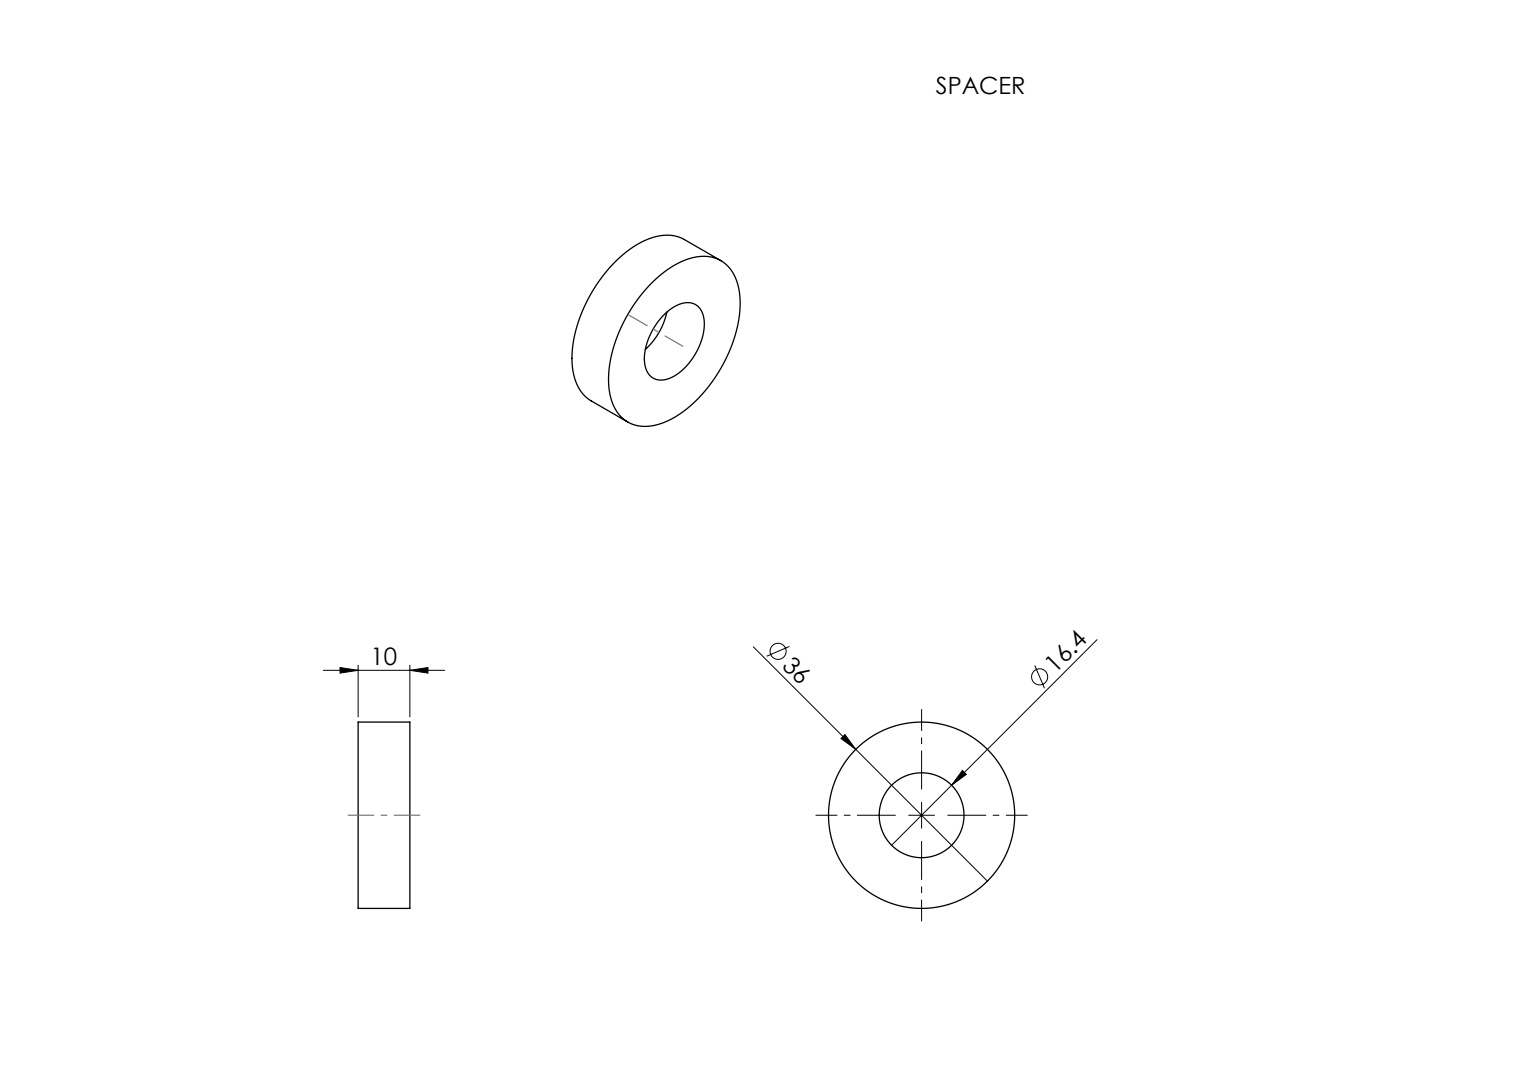
ISO-10303-21;
HEADER;
FILE_DESCRIPTION (('STEP AP214'),
    '1' );
FILE_NAME ('spacer.step',
    '2026-10-08T13:22:57',
    ( '' ),
    ( '' ),
    'SwSTEP 2.0',
    'SolidWorks 2026',
    '' );
FILE_SCHEMA (( 'AUTOMOTIVE_DESIGN' ));
ENDSEC;

DATA;
#27=LINE ( 'NONE', #8664, #6923 ) ;
#42=ORIENTED_EDGE ( 'NONE', *, *, #8056, .T. ) ;
#95=DIRECTION ( 'NONE',  ( 0.000000000000000000, 0.000000000000000000, 1.000000000000000000 ) ) ;
#147=MANIFOLD_SOLID_BREP ( 'Revolve1', #1849 ) ;
#192=( GEOMETRIC_REPRESENTATION_CONTEXT ( 3 ) GLOBAL_UNCERTAINTY_ASSIGNED_CONTEXT ( ( #920 ) ) GLOBAL_UNIT_ASSIGNED_CONTEXT ( ( #9393, #2545, #4632 ) ) REPRESENTATION_CONTEXT ( 'NONE', 'WORKASPACE' ) );
#245=CARTESIAN_POINT ( 'NONE',  ( 0.000000000000000000, 0.000000000000000000, 0.000000000000000000 ) ) ;
#270=( NAMED_UNIT ( * ) SI_UNIT ( $, .STERADIAN. ) SOLID_ANGLE_UNIT ( ) );
#321=ORIENTED_EDGE ( 'NONE', *, *, #2438, .F. ) ;
#336=AXIS2_PLACEMENT_3D ( 'NONE', #4011, #10212, #2306 ) ;
#339=AXIS2_PLACEMENT_3D ( 'NONE', #8130, #857, #5651 ) ;
#372=DIRECTION ( 'NONE',  ( -1.000000000000000000, 0.000000000000000000, -0.000000000000000000 ) ) ;
#398=UNCERTAINTY_MEASURE_WITH_UNIT (LENGTH_MEASURE( 1.000000000000000082E-05 ), #6272, 'distance_accuracy_value', 'NONE');
#440=DIRECTION ( 'NONE',  ( -1.000000000000000000, -0.000000000000000000, -0.000000000000000000 ) ) ;
#540=ORIENTED_EDGE ( 'NONE', *, *, #3932, .F. ) ;
#600=DIRECTION ( 'NONE',  ( -1.000000000000000000, -0.000000000000000000, -0.000000000000000000 ) ) ;
#614=SURFACE_STYLE_FILL_AREA ( #1388 ) ;
#808=EDGE_LOOP ( 'NONE', ( #8183, #7478, #5542, #1198 ) ) ;
#857=DIRECTION ( 'NONE',  ( -1.000000000000000000, -0.000000000000000000, -0.000000000000000000 ) ) ;
#920=UNCERTAINTY_MEASURE_WITH_UNIT (LENGTH_MEASURE( 1.000000000000000082E-05 ), #9393, 'distance_accuracy_value', 'NONE');
#1028=STYLED_ITEM ( 'NONE', ( #10063 ), #147 ) ;
#1052=DIRECTION ( 'NONE',  ( 0.000000000000000000, 0.000000000000000000, 1.000000000000000000 ) ) ;
#1099=DIRECTION ( 'NONE',  ( -1.000000000000000000, -0.000000000000000000, -0.000000000000000000 ) ) ;
#1144=FACE_BOUND ( 'NONE', #6677, .T. ) ;
#1198=ORIENTED_EDGE ( 'NONE', *, *, #7313, .F. ) ;
#1247=DIRECTION ( 'NONE',  ( 0.000000000000000000, 0.000000000000000000, 1.000000000000000000 ) ) ;
#1274=EDGE_CURVE ( 'NONE', #4587, #9073, #27, .T. ) ;
#1340=ADVANCED_FACE ( 'NONE', ( #3181 ), #7100, .F. ) ;
#1360=DIRECTION ( 'NONE',  ( -1.000000000000000000, -0.000000000000000000, -0.000000000000000000 ) ) ;
#1388=FILL_AREA_STYLE ('',( #8463 ) ) ;
#1479=CARTESIAN_POINT ( 'NONE',  ( -68.00000000000002842, 0.000000000000000000, 0.000000000000000000 ) ) ;
#1512=APPLICATION_CONTEXT ( 'automotive_design' ) ;
#1584=CARTESIAN_POINT ( 'NONE',  ( -68.00000000000002842, 1.004210375300829674E-15, -8.200000000000001066 ) ) ;
#1679=( GEOMETRIC_REPRESENTATION_CONTEXT ( 3 ) GLOBAL_UNCERTAINTY_ASSIGNED_CONTEXT ( ( #398 ) ) GLOBAL_UNIT_ASSIGNED_CONTEXT ( ( #6272, #5511, #4738 ) ) REPRESENTATION_CONTEXT ( 'NONE', 'WORKASPACE' ) );
#1745=ADVANCED_FACE ( 'NONE', ( #3549 ), #5914, .F. ) ;
#1824=VECTOR ( 'NONE', #440, 1000.000000000000000 ) ;
#1834=ORIENTED_EDGE ( 'NONE', *, *, #4659, .T. ) ;
#1849=CLOSED_SHELL ( 'NONE', ( #1340, #3482, #6215, #5630, #9440, #1745 ) ) ;
#1855=CIRCLE ( 'NONE', #7631, 8.200000000000001066 ) ;
#1888=ORIENTED_EDGE ( 'NONE', *, *, #1274, .F. ) ;
#1935=EDGE_LOOP ( 'NONE', ( #321, #4499, #6090, #10188 ) ) ;
#2035=DIRECTION ( 'NONE',  ( -1.000000000000000000, -0.000000000000000000, -0.000000000000000000 ) ) ;
#2086=CARTESIAN_POINT ( 'NONE',  ( -68.00000000000002842, 1.004210375300829674E-15, -8.200000000000001066 ) ) ;
#2115=EDGE_LOOP ( 'NONE', ( #8839, #9422, #2671, #1888 ) ) ;
#2143=CARTESIAN_POINT ( 'NONE',  ( -68.00000000000002842, 0.000000000000000000, 8.200000000000001066 ) ) ;
#2164=CIRCLE ( 'NONE', #9761, 18.00000000000000355 ) ;
#2201=AXIS2_PLACEMENT_3D ( 'NONE', #4351, #1360, #5991 ) ;
#2287=PLANE ( 'NONE',  #3033 ) ;
#2306=DIRECTION ( 'NONE',  ( 0.000000000000000000, 0.000000000000000000, 1.000000000000000000 ) ) ;
#2324=DIRECTION ( 'NONE',  ( -1.000000000000000000, -0.000000000000000000, -0.000000000000000000 ) ) ;
#2345=VECTOR ( 'NONE', #2035, 1000.000000000000000 ) ;
#2406=ORIENTED_EDGE ( 'NONE', *, *, #4728, .F. ) ;
#2433=EDGE_CURVE ( 'NONE', #6370, #5215, #9264, .T. ) ;
#2438=EDGE_CURVE ( 'NONE', #6370, #7745, #3691, .T. ) ;
#2446=PRODUCT_DEFINITION_FORMATION_WITH_SPECIFIED_SOURCE ( 'ANY', '', #3433, .NOT_KNOWN. ) ;
#2545=( NAMED_UNIT ( * ) PLANE_ANGLE_UNIT ( ) SI_UNIT ( $, .RADIAN. ) );
#2671=ORIENTED_EDGE ( 'NONE', *, *, #4371, .F. ) ;
#2804=DIRECTION ( 'NONE',  ( 0.000000000000000000, 0.000000000000000000, 1.000000000000000000 ) ) ;
#2872=ORIENTED_EDGE ( 'NONE', *, *, #2433, .T. ) ;
#2978=AXIS2_PLACEMENT_3D ( 'NONE', #5287, #8445, #2804 ) ;
#3033=AXIS2_PLACEMENT_3D ( 'NONE', #7911, #5431, #4566 ) ;
#3074=FILL_AREA_STYLE ('',( #4684 ) ) ;
#3082=AXIS2_PLACEMENT_3D ( 'NONE', #5180, #5837, #1247 ) ;
#3181=FACE_OUTER_BOUND ( 'NONE', #5847, .T. ) ;
#3247=ORIENTED_EDGE ( 'NONE', *, *, #2438, .T. ) ;
#3277=DIRECTION ( 'NONE',  ( -1.000000000000000000, -0.000000000000000000, -0.000000000000000000 ) ) ;
#3326=CARTESIAN_POINT ( 'NONE',  ( -58.00000000000001421, 2.204364238465235822E-15, -18.00000000000000355 ) ) ;
#3372=SURFACE_STYLE_USAGE ( .BOTH. , #6460 ) ;
#3374=VERTEX_POINT ( 'NONE', #3326 ) ;
#3433=PRODUCT ( 'spacer', 'spacer', '', ( #9046 ) ) ;
#3478=SHAPE_REPRESENTATION ( 'spacer', ( #3995 ), #6118 ) ;
#3482=ADVANCED_FACE ( 'NONE', ( #9886 ), #7451, .T. ) ;
#3531=CYLINDRICAL_SURFACE ( 'NONE', #7647, 18.00000000000000355 ) ;
#3549=FACE_OUTER_BOUND ( 'NONE', #1935, .T. ) ;
#3619=FACE_OUTER_BOUND ( 'NONE', #808, .T. ) ;
#3636=CARTESIAN_POINT ( 'NONE',  ( -58.00000000000001421, 0.000000000000000000, 18.00000000000000355 ) ) ;
#3691=LINE ( 'NONE', #2086, #1824 ) ;
#3716=EDGE_LOOP ( 'NONE', ( #5589, #6654 ) ) ;
#3761=SURFACE_SIDE_STYLE ('',( #614 ) ) ;
#3802=DIRECTION ( 'NONE',  ( 0.000000000000000000, 0.000000000000000000, 1.000000000000000000 ) ) ;
#3818=AXIS2_PLACEMENT_3D ( 'NONE', #1479, #600, #3802 ) ;
#3860=SHAPE_REPRESENTATION_RELATIONSHIP ( 'NONE' , 'NONE' ,  #3478, #8455 ) ;
#3876=EDGE_LOOP ( 'NONE', ( #540, #5439 ) ) ;
#3932=EDGE_CURVE ( 'NONE', #8337, #7745, #8041, .T. ) ;
#3995=AXIS2_PLACEMENT_3D ( 'NONE', #245, #8930, #7419 ) ;
#4011=CARTESIAN_POINT ( 'NONE',  ( -68.00000000000002842, 0.000000000000000000, 0.000000000000000000 ) ) ;
#4290=PLANE ( 'NONE',  #4803 ) ;
#4326=CARTESIAN_POINT ( 'NONE',  ( -68.00000000000002842, 0.000000000000000000, 0.000000000000000000 ) ) ;
#4351=CARTESIAN_POINT ( 'NONE',  ( -58.00000000000001421, 0.000000000000000000, 0.000000000000000000 ) ) ;
#4371=EDGE_CURVE ( 'NONE', #9073, #8249, #6614, .T. ) ;
#4418=LINE ( 'NONE', #5193, #2345 ) ;
#4423=PRODUCT_DEFINITION_CONTEXT ( 'detailed design', #6570, 'design' ) ;
#4440=SHAPE_DEFINITION_REPRESENTATION ( #5823, #3478 ) ;
#4499=ORIENTED_EDGE ( 'NONE', *, *, #8056, .F. ) ;
#4525=LINE ( 'NONE', #2143, #7149 ) ;
#4530=EDGE_CURVE ( 'NONE', #3374, #8249, #4418, .T. ) ;
#4566=DIRECTION ( 'NONE',  ( 0.000000000000000000, 0.000000000000000000, -1.000000000000000000 ) ) ;
#4587=VERTEX_POINT ( 'NONE', #3636 ) ;
#4632=( NAMED_UNIT ( * ) SI_UNIT ( $, .STERADIAN. ) SOLID_ANGLE_UNIT ( ) );
#4659=EDGE_CURVE ( 'NONE', #7745, #8337, #1855, .T. ) ;
#4684=FILL_AREA_STYLE_COLOUR ( '', #7288 ) ;
#4728=EDGE_CURVE ( 'NONE', #5215, #8337, #4525, .T. ) ;
#4738=( NAMED_UNIT ( * ) SI_UNIT ( $, .STERADIAN. ) SOLID_ANGLE_UNIT ( ) );
#4764=FACE_OUTER_BOUND ( 'NONE', #3716, .T. ) ;
#4784=DIRECTION ( 'NONE',  ( 0.000000000000000000, 0.000000000000000000, 1.000000000000000000 ) ) ;
#4803=AXIS2_PLACEMENT_3D ( 'NONE', #7447, #372, #9834 ) ;
#4968=CARTESIAN_POINT ( 'NONE',  ( -58.00000000000001421, 1.004210375300829674E-15, -8.200000000000001066 ) ) ;
#5025=ORIENTED_EDGE ( 'NONE', *, *, #5600, .F. ) ;
#5136=CARTESIAN_POINT ( 'NONE',  ( -68.00000000000002842, 2.204364238465235822E-15, -18.00000000000000355 ) ) ;
#5180=CARTESIAN_POINT ( 'NONE',  ( -68.00000000000002842, 0.000000000000000000, 0.000000000000000000 ) ) ;
#5193=CARTESIAN_POINT ( 'NONE',  ( -68.00000000000002842, 2.204364238465235822E-15, -18.00000000000000355 ) ) ;
#5215=VERTEX_POINT ( 'NONE', #8552 ) ;
#5220=CARTESIAN_POINT ( 'NONE',  ( -58.00000000000001421, 0.000000000000000000, 0.000000000000000000 ) ) ;
#5287=CARTESIAN_POINT ( 'NONE',  ( -58.00000000000001421, 0.000000000000000000, 0.000000000000000000 ) ) ;
#5431=DIRECTION ( 'NONE',  ( 1.000000000000000000, 0.000000000000000000, 0.000000000000000000 ) ) ;
#5439=ORIENTED_EDGE ( 'NONE', *, *, #4659, .F. ) ;
#5474=DIRECTION ( 'NONE',  ( 0.000000000000000000, 0.000000000000000000, 1.000000000000000000 ) ) ;
#5511=( NAMED_UNIT ( * ) PLANE_ANGLE_UNIT ( ) SI_UNIT ( $, .RADIAN. ) );
#5535=FACE_BOUND ( 'NONE', #3876, .T. ) ;
#5542=ORIENTED_EDGE ( 'NONE', *, *, #1274, .T. ) ;
#5589=ORIENTED_EDGE ( 'NONE', *, *, #4371, .T. ) ;
#5600=EDGE_CURVE ( 'NONE', #4587, #3374, #9304, .T. ) ;
#5630=ADVANCED_FACE ( 'NONE', ( #3619 ), #3531, .T. ) ;
#5651=DIRECTION ( 'NONE',  ( 0.000000000000000000, 0.000000000000000000, 1.000000000000000000 ) ) ;
#5689=( LENGTH_UNIT ( ) NAMED_UNIT ( * ) SI_UNIT ( .MILLI., .METRE. ) );
#5823=PRODUCT_DEFINITION_SHAPE ( 'NONE', 'NONE',  #7569 ) ;
#5837=DIRECTION ( 'NONE',  ( -1.000000000000000000, -0.000000000000000000, -0.000000000000000000 ) ) ;
#5840=DIRECTION ( 'NONE',  ( -1.000000000000000000, -0.000000000000000000, -0.000000000000000000 ) ) ;
#5847=EDGE_LOOP ( 'NONE', ( #9564, #3247, #1834, #2406 ) ) ;
#5914=CYLINDRICAL_SURFACE ( 'NONE', #6930, 8.200000000000001066 ) ;
#5991=DIRECTION ( 'NONE',  ( 0.000000000000000000, 0.000000000000000000, 1.000000000000000000 ) ) ;
#6089=MECHANICAL_DESIGN_GEOMETRIC_PRESENTATION_REPRESENTATION('',(#1028),#1679);
#6090=ORIENTED_EDGE ( 'NONE', *, *, #4728, .T. ) ;
#6118=( GEOMETRIC_REPRESENTATION_CONTEXT ( 3 ) GLOBAL_UNCERTAINTY_ASSIGNED_CONTEXT ( ( #9704 ) ) GLOBAL_UNIT_ASSIGNED_CONTEXT ( ( #5689, #8810, #270 ) ) REPRESENTATION_CONTEXT ( 'NONE', 'WORKASPACE' ) );
#6215=ADVANCED_FACE ( 'NONE', ( #5535, #4764 ), #2287, .F. ) ;
#6218=SURFACE_STYLE_FILL_AREA ( #3074 ) ;
#6272=( LENGTH_UNIT ( ) NAMED_UNIT ( * ) SI_UNIT ( .MILLI., .METRE. ) );
#6303=CARTESIAN_POINT ( 'NONE',  ( -68.00000000000002842, 0.000000000000000000, 18.00000000000000355 ) ) ;
#6370=VERTEX_POINT ( 'NONE', #4968 ) ;
#6407=PRESENTATION_STYLE_ASSIGNMENT (( #3372 ) ) ;
#6460=SURFACE_SIDE_STYLE ('',( #6218 ) ) ;
#6570=APPLICATION_CONTEXT ( 'automotive_design' ) ;
#6614=CIRCLE ( 'NONE', #8622, 18.00000000000000355 ) ;
#6654=ORIENTED_EDGE ( 'NONE', *, *, #7313, .T. ) ;
#6677=EDGE_LOOP ( 'NONE', ( #42, #2872 ) ) ;
#6708=CARTESIAN_POINT ( 'NONE',  ( -68.00000000000002842, 0.000000000000000000, 8.200000000000001066 ) ) ;
#6716=DIRECTION ( 'NONE',  ( -1.000000000000000000, -0.000000000000000000, -0.000000000000000000 ) ) ;
#6769=DIRECTION ( 'NONE',  ( 0.000000000000000000, 0.000000000000000000, 1.000000000000000000 ) ) ;
#6880=DIRECTION ( 'NONE',  ( -1.000000000000000000, -0.000000000000000000, -0.000000000000000000 ) ) ;
#6895=SURFACE_STYLE_USAGE ( .BOTH. , #3761 ) ;
#6923=VECTOR ( 'NONE', #3277, 1000.000000000000000 ) ;
#6930=AXIS2_PLACEMENT_3D ( 'NONE', #4326, #9087, #4784 ) ;
#7100=CYLINDRICAL_SURFACE ( 'NONE', #336, 8.200000000000001066 ) ;
#7103=CIRCLE ( 'NONE', #339, 8.200000000000001066 ) ;
#7149=VECTOR ( 'NONE', #6716, 1000.000000000000000 ) ;
#7178=DIRECTION ( 'NONE',  ( -1.000000000000000000, -0.000000000000000000, -0.000000000000000000 ) ) ;
#7215=AXIS2_PLACEMENT_3D ( 'NONE', #8417, #2324, #5474 ) ;
#7288=COLOUR_RGB ( '', 0.09019608, 0.27058824, 0.51372549) ;
#7313=EDGE_CURVE ( 'NONE', #8249, #9073, #7603, .T. ) ;
#7419=DIRECTION ( 'NONE',  ( 1.000000000000000000, 0.000000000000000000, 0.000000000000000000 ) ) ;
#7446=STYLED_ITEM ( 'NONE', ( #6407 ), #8455 ) ;
#7447=CARTESIAN_POINT ( 'NONE',  ( -58.00000000000001421, 8.200000000000001066, 0.000000000000000000 ) ) ;
#7451=CYLINDRICAL_SURFACE ( 'NONE', #3082, 18.00000000000000355 ) ;
#7478=ORIENTED_EDGE ( 'NONE', *, *, #9119, .T. ) ;
#7504=DIRECTION ( 'NONE',  ( 0.000000000000000000, 0.000000000000000000, 1.000000000000000000 ) ) ;
#7569=PRODUCT_DEFINITION ( 'UNKNOWN', '', #2446, #4423 ) ;
#7603=CIRCLE ( 'NONE', #3818, 18.00000000000000355 ) ;
#7631=AXIS2_PLACEMENT_3D ( 'NONE', #7682, #6880, #6769 ) ;
#7647=AXIS2_PLACEMENT_3D ( 'NONE', #9120, #5840, #7504 ) ;
#7682=CARTESIAN_POINT ( 'NONE',  ( -68.00000000000002842, 0.000000000000000000, 0.000000000000000000 ) ) ;
#7745=VERTEX_POINT ( 'NONE', #1584 ) ;
#7911=CARTESIAN_POINT ( 'NONE',  ( -68.00000000000002842, 8.200000000000001066, 0.000000000000000000 ) ) ;
#8041=CIRCLE ( 'NONE', #7215, 8.200000000000001066 ) ;
#8056=EDGE_CURVE ( 'NONE', #5215, #6370, #7103, .T. ) ;
#8130=CARTESIAN_POINT ( 'NONE',  ( -58.00000000000001421, 0.000000000000000000, 0.000000000000000000 ) ) ;
#8183=ORIENTED_EDGE ( 'NONE', *, *, #4530, .F. ) ;
#8215=FACE_OUTER_BOUND ( 'NONE', #9780, .T. ) ;
#8249=VERTEX_POINT ( 'NONE', #5136 ) ;
#8337=VERTEX_POINT ( 'NONE', #6708 ) ;
#8417=CARTESIAN_POINT ( 'NONE',  ( -68.00000000000002842, 0.000000000000000000, 0.000000000000000000 ) ) ;
#8445=DIRECTION ( 'NONE',  ( -1.000000000000000000, -0.000000000000000000, -0.000000000000000000 ) ) ;
#8455=ADVANCED_BREP_SHAPE_REPRESENTATION ( '', ( #147, #3995 ), #6118 ) ;
#8463=FILL_AREA_STYLE_COLOUR ( '', #8952 ) ;
#8552=CARTESIAN_POINT ( 'NONE',  ( -58.00000000000001421, 0.000000000000000000, 8.200000000000001066 ) ) ;
#8622=AXIS2_PLACEMENT_3D ( 'NONE', #8790, #7178, #95 ) ;
#8664=CARTESIAN_POINT ( 'NONE',  ( -68.00000000000002842, 0.000000000000000000, 18.00000000000000355 ) ) ;
#8777=MECHANICAL_DESIGN_GEOMETRIC_PRESENTATION_REPRESENTATION('',(#7446),#192);
#8790=CARTESIAN_POINT ( 'NONE',  ( -68.00000000000002842, 0.000000000000000000, 0.000000000000000000 ) ) ;
#8810=( NAMED_UNIT ( * ) PLANE_ANGLE_UNIT ( ) SI_UNIT ( $, .RADIAN. ) );
#8839=ORIENTED_EDGE ( 'NONE', *, *, #5600, .T. ) ;
#8930=DIRECTION ( 'NONE',  ( 0.000000000000000000, 0.000000000000000000, 1.000000000000000000 ) ) ;
#8952=COLOUR_RGB ( '', 0.09019608, 0.27058824, 0.51372549) ;
#9046=PRODUCT_CONTEXT ( 'NONE', #1512, 'mechanical' ) ;
#9073=VERTEX_POINT ( 'NONE', #6303 ) ;
#9087=DIRECTION ( 'NONE',  ( -1.000000000000000000, -0.000000000000000000, -0.000000000000000000 ) ) ;
#9119=EDGE_CURVE ( 'NONE', #3374, #4587, #2164, .T. ) ;
#9120=CARTESIAN_POINT ( 'NONE',  ( -68.00000000000002842, 0.000000000000000000, 0.000000000000000000 ) ) ;
#9264=CIRCLE ( 'NONE', #2978, 8.200000000000001066 ) ;
#9304=CIRCLE ( 'NONE', #2201, 18.00000000000000355 ) ;
#9382=ORIENTED_EDGE ( 'NONE', *, *, #9119, .F. ) ;
#9393=( LENGTH_UNIT ( ) NAMED_UNIT ( * ) SI_UNIT ( .MILLI., .METRE. ) );
#9422=ORIENTED_EDGE ( 'NONE', *, *, #4530, .T. ) ;
#9440=ADVANCED_FACE ( 'NONE', ( #8215, #1144 ), #4290, .F. ) ;
#9564=ORIENTED_EDGE ( 'NONE', *, *, #2433, .F. ) ;
#9704=UNCERTAINTY_MEASURE_WITH_UNIT (LENGTH_MEASURE( 1.000000000000000082E-05 ), #5689, 'distance_accuracy_value', 'NONE');
#9761=AXIS2_PLACEMENT_3D ( 'NONE', #5220, #1099, #1052 ) ;
#9780=EDGE_LOOP ( 'NONE', ( #5025, #9382 ) ) ;
#9834=DIRECTION ( 'NONE',  ( -0.000000000000000000, 0.000000000000000000, 1.000000000000000000 ) ) ;
#9886=FACE_OUTER_BOUND ( 'NONE', #2115, .T. ) ;
#10063=PRESENTATION_STYLE_ASSIGNMENT (( #6895 ) ) ;
#10188=ORIENTED_EDGE ( 'NONE', *, *, #3932, .T. ) ;
#10212=DIRECTION ( 'NONE',  ( -1.000000000000000000, -0.000000000000000000, -0.000000000000000000 ) ) ;
ENDSEC;
END-ISO-10303-21;
